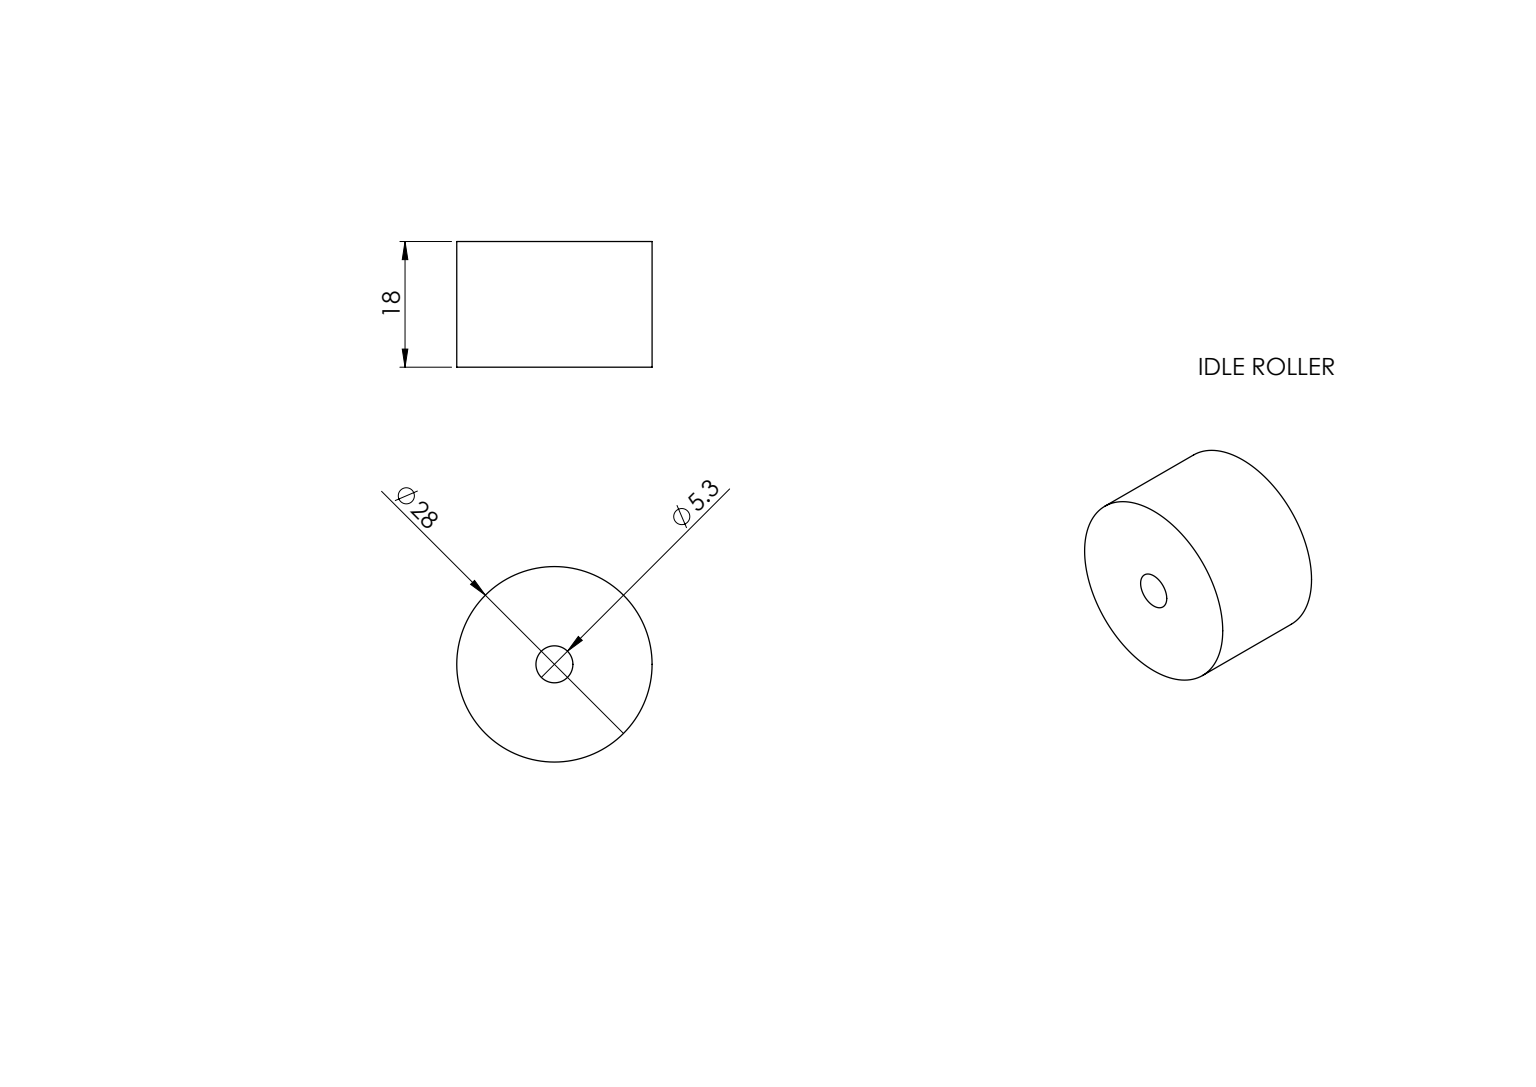
ISO-10303-21;
HEADER;
FILE_DESCRIPTION (('STEP AP214'),
    '1' );
FILE_NAME ('idle roller.step',
    '2026-10-31T03:44:21',
    ( '' ),
    ( '' ),
    'SwSTEP 2.0',
    'SolidWorks 2026',
    '' );
FILE_SCHEMA (( 'AUTOMOTIVE_DESIGN' ));
ENDSEC;

DATA;
#113=( NAMED_UNIT ( * ) SI_UNIT ( $, .STERADIAN. ) SOLID_ANGLE_UNIT ( ) );
#203=DIRECTION ( 'NONE',  ( -0.000000000000000000, -0.000000000000000000, 1.000000000000000000 ) ) ;
#498=CARTESIAN_POINT ( 'NONE',  ( 1.925929944387235853E-31, 15.00000000000001599, -9.000000000000000000 ) ) ;
#623=CYLINDRICAL_SURFACE ( 'NONE', #10678, 2.649999999999988365 ) ;
#633=ORIENTED_EDGE ( 'NONE', *, *, #4119, .T. ) ;
#648=AXIS2_PLACEMENT_3D ( 'NONE', #17257, #13019, #13119 ) ;
#881=VECTOR ( 'NONE', #3136, 1000.000000000000000 ) ;
#896=AXIS2_PLACEMENT_3D ( 'NONE', #10269, #16272, #2847 ) ;
#1000=DIRECTION ( 'NONE',  ( 1.000000000000000000, 0.000000000000000000, 0.000000000000000000 ) ) ;
#1104=ORIENTED_EDGE ( 'NONE', *, *, #14646, .F. ) ;
#1317=EDGE_CURVE ( 'NONE', #4060, #2011, #16539, .T. ) ;
#1341=ORIENTED_EDGE ( 'NONE', *, *, #16606, .F. ) ;
#1362=FACE_OUTER_BOUND ( 'NONE', #9886, .T. ) ;
#1532=( GEOMETRIC_REPRESENTATION_CONTEXT ( 3 ) GLOBAL_UNCERTAINTY_ASSIGNED_CONTEXT ( ( #15377 ) ) GLOBAL_UNIT_ASSIGNED_CONTEXT ( ( #4479, #3113, #14956 ) ) REPRESENTATION_CONTEXT ( 'NONE', 'WORKASPACE' ) );
#1586=( NAMED_UNIT ( * ) PLANE_ANGLE_UNIT ( ) SI_UNIT ( $, .RADIAN. ) );
#1672=UNCERTAINTY_MEASURE_WITH_UNIT (LENGTH_MEASURE( 1.000000000000000082E-05 ), #16777, 'distance_accuracy_value', 'NONE');
#1765=CARTESIAN_POINT ( 'NONE',  ( -2.649999999999989697, 15.00000000000001599, -9.000000000000001776 ) ) ;
#1821=ORIENTED_EDGE ( 'NONE', *, *, #8177, .F. ) ;
#2011=VERTEX_POINT ( 'NONE', #14697 ) ;
#2027=AXIS2_PLACEMENT_3D ( 'NONE', #17172, #6855, #12746 ) ;
#2410=ORIENTED_EDGE ( 'NONE', *, *, #4119, .F. ) ;
#2485=CIRCLE ( 'NONE', #5285, 14.00000000000000000 ) ;
#2534=DIRECTION ( 'NONE',  ( -0.000000000000000000, -0.000000000000000000, -1.000000000000000000 ) ) ;
#2706=ADVANCED_FACE ( 'NONE', ( #18078, #9137 ), #4740, .T. ) ;
#2847=DIRECTION ( 'NONE',  ( 1.000000000000000000, 0.000000000000000000, 0.000000000000000000 ) ) ;
#2871=CARTESIAN_POINT ( 'NONE',  ( 0.000000000000000000, 0.000000000000000000, 0.000000000000000000 ) ) ;
#2987=CARTESIAN_POINT ( 'NONE',  ( 14.00000000000000000, 15.00000000000001776, 9.000000000000000000 ) ) ;
#3056=CARTESIAN_POINT ( 'NONE',  ( 1.925929944387235853E-31, 15.00000000000001599, -9.000000000000001776 ) ) ;
#3113=( NAMED_UNIT ( * ) PLANE_ANGLE_UNIT ( ) SI_UNIT ( $, .RADIAN. ) );
#3136=DIRECTION ( 'NONE',  ( -0.000000000000000000, -0.000000000000000000, 1.000000000000000000 ) ) ;
#3341=SHAPE_REPRESENTATION_RELATIONSHIP ( 'NONE' , 'NONE' ,  #4676, #16200 ) ;
#3349=LINE ( 'NONE', #4908, #16918 ) ;
#3401=( GEOMETRIC_REPRESENTATION_CONTEXT ( 3 ) GLOBAL_UNCERTAINTY_ASSIGNED_CONTEXT ( ( #4982 ) ) GLOBAL_UNIT_ASSIGNED_CONTEXT ( ( #9123, #1586, #113 ) ) REPRESENTATION_CONTEXT ( 'NONE', 'WORKASPACE' ) );
#3411=ORIENTED_EDGE ( 'NONE', *, *, #15144, .T. ) ;
#3439=SURFACE_SIDE_STYLE ('',( #16874 ) ) ;
#3461=ADVANCED_FACE ( 'NONE', ( #4560 ), #12188, .T. ) ;
#3469=AXIS2_PLACEMENT_3D ( 'NONE', #14213, #14315, #1000 ) ;
#3501=AXIS2_PLACEMENT_3D ( 'NONE', #8941, #15121, #7664 ) ;
#3543=DIRECTION ( 'NONE',  ( 0.000000000000000000, 0.000000000000000000, 1.000000000000000000 ) ) ;
#3704=VERTEX_POINT ( 'NONE', #14327 ) ;
#3780=ORIENTED_EDGE ( 'NONE', *, *, #16013, .T. ) ;
#3782=ORIENTED_EDGE ( 'NONE', *, *, #16606, .T. ) ;
#4031=COLOUR_RGB ( '',0.8941176470588234615, 0.8941176470588234615, 0.8941176470588234615 ) ;
#4060=VERTEX_POINT ( 'NONE', #15593 ) ;
#4115=ORIENTED_EDGE ( 'NONE', *, *, #19379, .F. ) ;
#4118=ORIENTED_EDGE ( 'NONE', *, *, #4188, .F. ) ;
#4119=EDGE_CURVE ( 'NONE', #7193, #15477, #17370, .T. ) ;
#4134=ORIENTED_EDGE ( 'NONE', *, *, #13706, .F. ) ;
#4188=EDGE_CURVE ( 'NONE', #3704, #9229, #18945, .T. ) ;
#4251=CARTESIAN_POINT ( 'NONE',  ( -14.00000000000000000, 15.00000000000001599, 9.000000000000000000 ) ) ;
#4349=LINE ( 'NONE', #2987, #10915 ) ;
#4412=ORIENTED_EDGE ( 'NONE', *, *, #1317, .T. ) ;
#4479=( LENGTH_UNIT ( ) NAMED_UNIT ( * ) SI_UNIT ( .MILLI., .METRE. ) );
#4560=FACE_OUTER_BOUND ( 'NONE', #18353, .T. ) ;
#4647=VERTEX_POINT ( 'NONE', #1765 ) ;
#4676=SHAPE_REPRESENTATION ( 'idle roller', ( #10359 ), #12782 ) ;
#4740=PLANE ( 'NONE',  #3501 ) ;
#4882=DIRECTION ( 'NONE',  ( 0.000000000000000000, 0.000000000000000000, 1.000000000000000000 ) ) ;
#4908=CARTESIAN_POINT ( 'NONE',  ( 2.649999999999988365, 15.00000000000001599, 15.00000000000000000 ) ) ;
#4982=UNCERTAINTY_MEASURE_WITH_UNIT (LENGTH_MEASURE( 1.000000000000000082E-05 ), #9123, 'distance_accuracy_value', 'NONE');
#5006=DIRECTION ( 'NONE',  ( 1.000000000000000000, 0.000000000000000000, 0.000000000000000000 ) ) ;
#5285=AXIS2_PLACEMENT_3D ( 'NONE', #7909, #4882, #18137 ) ;
#5377=PLANE ( 'NONE',  #648 ) ;
#5463=CARTESIAN_POINT ( 'NONE',  ( 1.925929944387235853E-31, 15.00000000000001599, -9.000000000000000000 ) ) ;
#5629=AXIS2_PLACEMENT_3D ( 'NONE', #3056, #203, #15550 ) ;
#5674=DIRECTION ( 'NONE',  ( 1.000000000000000000, 0.000000000000000000, 0.000000000000000000 ) ) ;
#6169=ADVANCED_FACE ( 'NONE', ( #12830, #15971 ), #5377, .F. ) ;
#6187=CIRCLE ( 'NONE', #9599, 14.00000000000000000 ) ;
#6515=ORIENTED_EDGE ( 'NONE', *, *, #14646, .T. ) ;
#6600=CARTESIAN_POINT ( 'NONE',  ( 1.925929944387235853E-31, 15.00000000000001599, 15.00000000000000000 ) ) ;
#6612=PRODUCT_DEFINITION ( 'UNKNOWN', '', #16072, #14991 ) ;
#6744=ADVANCED_FACE ( 'NONE', ( #15753 ), #6918, .T. ) ;
#6855=DIRECTION ( 'NONE',  ( 0.000000000000000000, 0.000000000000000000, 1.000000000000000000 ) ) ;
#6918=CYLINDRICAL_SURFACE ( 'NONE', #12860, 14.00000000000000000 ) ;
#7014=DIRECTION ( 'NONE',  ( -1.000000000000000000, 0.000000000000000000, 0.000000000000000000 ) ) ;
#7087=DIRECTION ( 'NONE',  ( -0.000000000000000000, -0.000000000000000000, -1.000000000000000000 ) ) ;
#7148=MECHANICAL_DESIGN_GEOMETRIC_PRESENTATION_REPRESENTATION('',(#15925),#3401);
#7193=VERTEX_POINT ( 'NONE', #11392 ) ;
#7264=ADVANCED_FACE ( 'NONE', ( #14039 ), #623, .F. ) ;
#7320=AXIS2_PLACEMENT_3D ( 'NONE', #9054, #10717, #15042 ) ;
#7335=CYLINDRICAL_SURFACE ( 'NONE', #14657, 2.649999999999988365 ) ;
#7336=AXIS2_PLACEMENT_3D ( 'NONE', #498, #3543, #5006 ) ;
#7367=CARTESIAN_POINT ( 'NONE',  ( 2.649999999999988365, 15.00000000000001599, 9.000000000000000000 ) ) ;
#7435=CARTESIAN_POINT ( 'NONE',  ( 1.925929944387235853E-31, 15.00000000000001599, 15.00000000000000000 ) ) ;
#7664=DIRECTION ( 'NONE',  ( 1.000000000000000000, 0.000000000000000000, -0.000000000000000000 ) ) ;
#7909=CARTESIAN_POINT ( 'NONE',  ( 1.925929944387235853E-31, 15.00000000000001599, 9.000000000000000000 ) ) ;
#8067=ORIENTED_EDGE ( 'NONE', *, *, #19379, .T. ) ;
#8177=EDGE_CURVE ( 'NONE', #15477, #7193, #6187, .T. ) ;
#8732=STYLED_ITEM('',(#19454),#15430);
#8834=DIRECTION ( 'NONE',  ( 0.000000000000000000, 0.000000000000000000, 1.000000000000000000 ) ) ;
#8941=CARTESIAN_POINT ( 'NONE',  ( 1.925929944387235853E-31, 15.00000000000001599, 9.000000000000000000 ) ) ;
#8973=CARTESIAN_POINT ( 'NONE',  ( -14.00000000000000000, 15.00000000000001599, -9.000000000000000000 ) ) ;
#8992=AXIS2_PLACEMENT_3D ( 'NONE', #16112, #17490, #11385 ) ;
#9054=CARTESIAN_POINT ( 'NONE',  ( 1.925929944387235853E-31, 15.00000000000001599, 9.000000000000000000 ) ) ;
#9104=CIRCLE ( 'NONE', #3469, 2.649999999999988365 ) ;
#9123=( LENGTH_UNIT ( ) NAMED_UNIT ( * ) SI_UNIT ( .MILLI., .METRE. ) );
#9137=FACE_OUTER_BOUND ( 'NONE', #11308, .T. ) ;
#9229=VERTEX_POINT ( 'NONE', #7367 ) ;
#9334=CIRCLE ( 'NONE', #896, 2.649999999999989697 ) ;
#9383=EDGE_LOOP ( 'NONE', ( #13602, #10458, #3782, #8067 ) ) ;
#9401=SURFACE_STYLE_USAGE ( .BOTH. , #3439 ) ;
#9599=AXIS2_PLACEMENT_3D ( 'NONE', #5463, #11050, #18828 ) ;
#9750=PRODUCT_DEFINITION_SHAPE ( 'NONE', 'NONE',  #6612 ) ;
#9860=EDGE_LOOP ( 'NONE', ( #13002, #3780, #633, #1104 ) ) ;
#9886=EDGE_LOOP ( 'NONE', ( #18782, #16370, #13693, #1341 ) ) ;
#9979=ORIENTED_EDGE ( 'NONE', *, *, #8177, .T. ) ;
#10104=VECTOR ( 'NONE', #7087, 1000.000000000000000 ) ;
#10146=EDGE_LOOP ( 'NONE', ( #14399, #3411 ) ) ;
#10220=ORIENTED_EDGE ( 'NONE', *, *, #13706, .T. ) ;
#10269=CARTESIAN_POINT ( 'NONE',  ( 1.925929944387235853E-31, 15.00000000000001599, -9.000000000000001776 ) ) ;
#10359=AXIS2_PLACEMENT_3D ( 'NONE', #2871, #8834, #16191 ) ;
#10458=ORIENTED_EDGE ( 'NONE', *, *, #18185, .F. ) ;
#10555=LINE ( 'NONE', #17742, #881 ) ;
#10678=AXIS2_PLACEMENT_3D ( 'NONE', #6600, #18592, #13330 ) ;
#10717=DIRECTION ( 'NONE',  ( -0.000000000000000000, -0.000000000000000000, -1.000000000000000000 ) ) ;
#10868=FILL_AREA_STYLE_COLOUR ( '', #4031 ) ;
#10915=VECTOR ( 'NONE', #19189, 1000.000000000000000 ) ;
#11050=DIRECTION ( 'NONE',  ( 0.000000000000000000, 0.000000000000000000, 1.000000000000000000 ) ) ;
#11260=VERTEX_POINT ( 'NONE', #19116 ) ;
#11308=EDGE_LOOP ( 'NONE', ( #10220, #4412 ) ) ;
#11385=DIRECTION ( 'NONE',  ( 1.000000000000000000, 0.000000000000000000, 0.000000000000000000 ) ) ;
#11392=CARTESIAN_POINT ( 'NONE',  ( 14.00000000000000000, 15.00000000000001776, -9.000000000000000000 ) ) ;
#11737=DIRECTION ( 'NONE',  ( -0.000000000000000000, -0.000000000000000000, 1.000000000000000000 ) ) ;
#11785=LINE ( 'NONE', #4251, #10104 ) ;
#12188=CYLINDRICAL_SURFACE ( 'NONE', #7320, 14.00000000000000000 ) ;
#12714=EDGE_LOOP ( 'NONE', ( #4115, #4118 ) ) ;
#12746=DIRECTION ( 'NONE',  ( 1.000000000000000000, 0.000000000000000000, 0.000000000000000000 ) ) ;
#12782=( GEOMETRIC_REPRESENTATION_CONTEXT ( 3 ) GLOBAL_UNCERTAINTY_ASSIGNED_CONTEXT ( ( #1672 ) ) GLOBAL_UNIT_ASSIGNED_CONTEXT ( ( #16777, #15197, #13818 ) ) REPRESENTATION_CONTEXT ( 'NONE', 'WORKASPACE' ) );
#12830=FACE_BOUND ( 'NONE', #10146, .T. ) ;
#12860=AXIS2_PLACEMENT_3D ( 'NONE', #15845, #2534, #7014 ) ;
#12948=ORIENTED_EDGE ( 'NONE', *, *, #16013, .F. ) ;
#13002=ORIENTED_EDGE ( 'NONE', *, *, #1317, .F. ) ;
#13019=DIRECTION ( 'NONE',  ( 0.000000000000000000, 0.000000000000000000, 1.000000000000000000 ) ) ;
#13052=PRODUCT ( 'idle roller', 'idle roller', '', ( #13726 ) ) ;
#13119=DIRECTION ( 'NONE',  ( 1.000000000000000000, 0.000000000000000000, -0.000000000000000000 ) ) ;
#13330=DIRECTION ( 'NONE',  ( 1.000000000000000000, 0.000000000000000000, 0.000000000000000000 ) ) ;
#13482=ADVANCED_FACE ( 'NONE', ( #1362 ), #7335, .F. ) ;
#13584=EDGE_CURVE ( 'NONE', #4647, #3704, #10555, .T. ) ;
#13602=ORIENTED_EDGE ( 'NONE', *, *, #13584, .F. ) ;
#13693=ORIENTED_EDGE ( 'NONE', *, *, #4188, .T. ) ;
#13706=EDGE_CURVE ( 'NONE', #2011, #4060, #2485, .T. ) ;
#13726=PRODUCT_CONTEXT ( 'NONE', #14889, 'mechanical' ) ;
#13818=( NAMED_UNIT ( * ) SI_UNIT ( $, .STERADIAN. ) SOLID_ANGLE_UNIT ( ) );
#14039=FACE_OUTER_BOUND ( 'NONE', #9383, .T. ) ;
#14072=CIRCLE ( 'NONE', #5629, 2.649999999999989697 ) ;
#14213=CARTESIAN_POINT ( 'NONE',  ( 1.925929944387235853E-31, 15.00000000000001599, 9.000000000000000000 ) ) ;
#14315=DIRECTION ( 'NONE',  ( 0.000000000000000000, 0.000000000000000000, 1.000000000000000000 ) ) ;
#14327=CARTESIAN_POINT ( 'NONE',  ( -2.649999999999988365, 15.00000000000001599, 9.000000000000000000 ) ) ;
#14399=ORIENTED_EDGE ( 'NONE', *, *, #18185, .T. ) ;
#14646=EDGE_CURVE ( 'NONE', #2011, #15477, #11785, .T. ) ;
#14657=AXIS2_PLACEMENT_3D ( 'NONE', #7435, #11737, #5674 ) ;
#14697=CARTESIAN_POINT ( 'NONE',  ( -14.00000000000000000, 15.00000000000001599, 9.000000000000000000 ) ) ;
#14889=APPLICATION_CONTEXT ( 'automotive_design' ) ;
#14956=( NAMED_UNIT ( * ) SI_UNIT ( $, .STERADIAN. ) SOLID_ANGLE_UNIT ( ) );
#14991=PRODUCT_DEFINITION_CONTEXT ( 'detailed design', #16692, 'design' ) ;
#15042=DIRECTION ( 'NONE',  ( -1.000000000000000000, 0.000000000000000000, 0.000000000000000000 ) ) ;
#15121=DIRECTION ( 'NONE',  ( 0.000000000000000000, 0.000000000000000000, 1.000000000000000000 ) ) ;
#15144=EDGE_CURVE ( 'NONE', #4647, #11260, #9334, .T. ) ;
#15197=( NAMED_UNIT ( * ) PLANE_ANGLE_UNIT ( ) SI_UNIT ( $, .RADIAN. ) );
#15199=SHAPE_DEFINITION_REPRESENTATION ( #9750, #4676 ) ;
#15377=UNCERTAINTY_MEASURE_WITH_UNIT (LENGTH_MEASURE( 1.000000000000000082E-05 ), #4479, 'distance_accuracy_value', 'NONE');
#15430=MANIFOLD_SOLID_BREP ( 'M5 Clearance Hole1', #18084 ) ;
#15477=VERTEX_POINT ( 'NONE', #8973 ) ;
#15550=DIRECTION ( 'NONE',  ( 1.000000000000000000, 0.000000000000000000, 0.000000000000000000 ) ) ;
#15593=CARTESIAN_POINT ( 'NONE',  ( 14.00000000000000000, 15.00000000000001776, 9.000000000000000000 ) ) ;
#15753=FACE_OUTER_BOUND ( 'NONE', #9860, .T. ) ;
#15845=CARTESIAN_POINT ( 'NONE',  ( 1.925929944387235853E-31, 15.00000000000001599, 9.000000000000000000 ) ) ;
#15925=STYLED_ITEM ( 'NONE', ( #16979 ), #16200 ) ;
#15971=FACE_OUTER_BOUND ( 'NONE', #19082, .T. ) ;
#16013=EDGE_CURVE ( 'NONE', #4060, #7193, #4349, .T. ) ;
#16072=PRODUCT_DEFINITION_FORMATION_WITH_SPECIFIED_SOURCE ( 'ANY', '', #13052, .NOT_KNOWN. ) ;
#16112=CARTESIAN_POINT ( 'NONE',  ( 1.925929944387235853E-31, 15.00000000000001599, 9.000000000000000000 ) ) ;
#16191=DIRECTION ( 'NONE',  ( 1.000000000000000000, 0.000000000000000000, 0.000000000000000000 ) ) ;
#16200=ADVANCED_BREP_SHAPE_REPRESENTATION ( '', ( #15430, #10359 ), #12782 ) ;
#16262=MECHANICAL_DESIGN_GEOMETRIC_PRESENTATION_REPRESENTATION('',(#8732),#1532);
#16272=DIRECTION ( 'NONE',  ( -0.000000000000000000, -0.000000000000000000, 1.000000000000000000 ) ) ;
#16370=ORIENTED_EDGE ( 'NONE', *, *, #13584, .T. ) ;
#16539=CIRCLE ( 'NONE', #8992, 14.00000000000000000 ) ;
#16585=FILL_AREA_STYLE ('',( #10868 ) ) ;
#16592=DIRECTION ( 'NONE',  ( -0.000000000000000000, -0.000000000000000000, 1.000000000000000000 ) ) ;
#16606=EDGE_CURVE ( 'NONE', #11260, #9229, #3349, .T. ) ;
#16692=APPLICATION_CONTEXT ( 'automotive_design' ) ;
#16777=( LENGTH_UNIT ( ) NAMED_UNIT ( * ) SI_UNIT ( .MILLI., .METRE. ) );
#16874=SURFACE_STYLE_FILL_AREA ( #16585 ) ;
#16918=VECTOR ( 'NONE', #16592, 1000.000000000000000 ) ;
#16979=PRESENTATION_STYLE_ASSIGNMENT (( #9401 ) ) ;
#17172=CARTESIAN_POINT ( 'NONE',  ( 1.925929944387235853E-31, 15.00000000000001599, 9.000000000000000000 ) ) ;
#17257=CARTESIAN_POINT ( 'NONE',  ( 1.925929944387235853E-31, 15.00000000000001599, -9.000000000000000000 ) ) ;
#17370=CIRCLE ( 'NONE', #7336, 14.00000000000000000 ) ;
#17490=DIRECTION ( 'NONE',  ( 0.000000000000000000, 0.000000000000000000, 1.000000000000000000 ) ) ;
#17742=CARTESIAN_POINT ( 'NONE',  ( -2.649999999999988365, 15.00000000000001599, 15.00000000000000000 ) ) ;
#18078=FACE_BOUND ( 'NONE', #12714, .T. ) ;
#18084=CLOSED_SHELL ( 'NONE', ( #13482, #6744, #3461, #2706, #6169, #7264 ) ) ;
#18137=DIRECTION ( 'NONE',  ( 1.000000000000000000, 0.000000000000000000, 0.000000000000000000 ) ) ;
#18185=EDGE_CURVE ( 'NONE', #11260, #4647, #14072, .T. ) ;
#18353=EDGE_LOOP ( 'NONE', ( #12948, #4134, #6515, #9979 ) ) ;
#18592=DIRECTION ( 'NONE',  ( -0.000000000000000000, -0.000000000000000000, 1.000000000000000000 ) ) ;
#18782=ORIENTED_EDGE ( 'NONE', *, *, #15144, .F. ) ;
#18828=DIRECTION ( 'NONE',  ( 1.000000000000000000, 0.000000000000000000, 0.000000000000000000 ) ) ;
#18945=CIRCLE ( 'NONE', #2027, 2.649999999999988365 ) ;
#19082=EDGE_LOOP ( 'NONE', ( #1821, #2410 ) ) ;
#19116=CARTESIAN_POINT ( 'NONE',  ( 2.649999999999989697, 15.00000000000001599, -9.000000000000001776 ) ) ;
#19189=DIRECTION ( 'NONE',  ( -0.000000000000000000, -0.000000000000000000, -1.000000000000000000 ) ) ;
#19379=EDGE_CURVE ( 'NONE', #9229, #3704, #9104, .T. ) ;
#19448=COLOUR_RGB('Light Blue',0.38,0.62,0.78);
#19449=FILL_AREA_STYLE_COLOUR('',#19448);
#19450=FILL_AREA_STYLE('',(#19449));
#19451=SURFACE_STYLE_FILL_AREA(#19450);
#19452=SURFACE_SIDE_STYLE('',(#19451));
#19453=SURFACE_STYLE_USAGE(.BOTH.,#19452);
#19454=PRESENTATION_STYLE_ASSIGNMENT((#19453));
ENDSEC;
END-ISO-10303-21;
